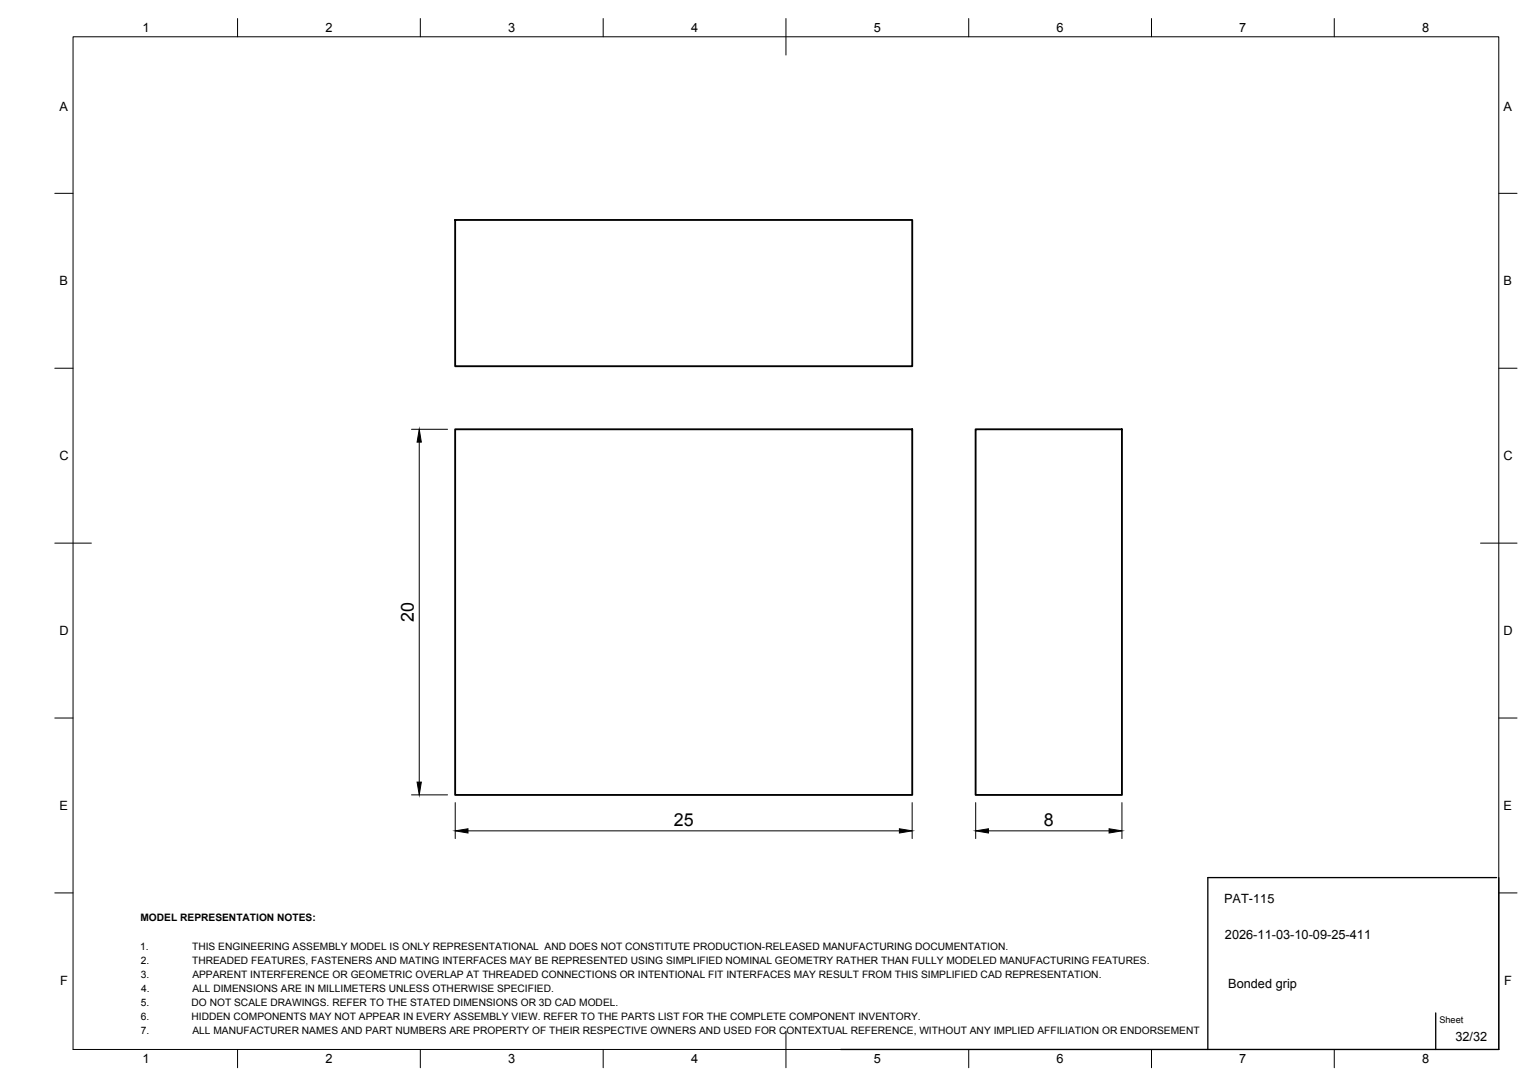
ISO-10303-21;
HEADER;
/* Generated by software containing ST-Developer
 * from STEP Tools, Inc. (www.steptools.com) 
 */

FILE_DESCRIPTION(
/* description */ ('Union bypass pipe loop'),
/* implementation_level */ '2;1');

FILE_NAME(
/* name */ 'Bonded grip.step',
/* time_stamp */ '2026-10-27T21:00:29-07:00',
/* author */ (''),
/* organization */ (''),
/* preprocessor_version */ 'ST-DEVELOPER v20.2',
/* originating_system */ 'Autodesk Translation Framework v15.17.0.0',
/* authorisation */ '');

FILE_SCHEMA (('AUTOMOTIVE_DESIGN { 1 0 10303 214 3 1 1 }'));
ENDSEC;

DATA;
#10=MECHANICAL_DESIGN_GEOMETRIC_PRESENTATION_REPRESENTATION('',(#475),#10095);
#411=SHAPE_REPRESENTATION_RELATIONSHIP('SRR','None',#10281,#443);
#443=ADVANCED_BREP_SHAPE_REPRESENTATION('',(#504),#10093);
#475=STYLED_ITEM('',(#10507),#504);
#504=MANIFOLD_SOLID_BREP('Body1',#5549);
#818=PLANE('',#6581);
#819=PLANE('',#6582);
#820=PLANE('',#6583);
#821=PLANE('',#6584);
#822=PLANE('',#6585);
#823=PLANE('',#6586);
#1145=FACE_OUTER_BOUND('',#1600,.T.);
#1146=FACE_OUTER_BOUND('',#1601,.T.);
#1147=FACE_OUTER_BOUND('',#1602,.T.);
#1148=FACE_OUTER_BOUND('',#1603,.T.);
#1149=FACE_OUTER_BOUND('',#1604,.T.);
#1150=FACE_OUTER_BOUND('',#1605,.T.);
#1600=EDGE_LOOP('',(#4996,#4997,#4998,#4999));
#1601=EDGE_LOOP('',(#5000,#5001,#5002,#5003));
#1602=EDGE_LOOP('',(#5004,#5005,#5006,#5007));
#1603=EDGE_LOOP('',(#5008,#5009,#5010,#5011));
#1604=EDGE_LOOP('',(#5012,#5013,#5014,#5015));
#1605=EDGE_LOOP('',(#5016,#5017,#5018,#5019));
#1964=LINE('',#9925,#2340);
#1965=LINE('',#9927,#2341);
#1966=LINE('',#9929,#2342);
#1967=LINE('',#9930,#2343);
#1968=LINE('',#9933,#2344);
#1969=LINE('',#9935,#2345);
#1970=LINE('',#9936,#2346);
#1971=LINE('',#9939,#2347);
#1972=LINE('',#9941,#2348);
#1973=LINE('',#9942,#2349);
#1974=LINE('',#9944,#2350);
#1975=LINE('',#9945,#2351);
#2340=VECTOR('',#8314,1.);
#2341=VECTOR('',#8315,1.);
#2342=VECTOR('',#8316,1.);
#2343=VECTOR('',#8317,1.);
#2344=VECTOR('',#8320,1.);
#2345=VECTOR('',#8321,1.);
#2346=VECTOR('',#8322,1.);
#2347=VECTOR('',#8325,1.);
#2348=VECTOR('',#8326,1.);
#2349=VECTOR('',#8327,1.);
#2350=VECTOR('',#8330,1.);
#2351=VECTOR('',#8331,1.);
#3040=VERTEX_POINT('',#9923);
#3041=VERTEX_POINT('',#9924);
#3042=VERTEX_POINT('',#9926);
#3043=VERTEX_POINT('',#9928);
#3044=VERTEX_POINT('',#9932);
#3045=VERTEX_POINT('',#9934);
#3046=VERTEX_POINT('',#9938);
#3047=VERTEX_POINT('',#9940);
#3696=EDGE_CURVE('',#3040,#3041,#1964,.T.);
#3697=EDGE_CURVE('',#3041,#3042,#1965,.T.);
#3698=EDGE_CURVE('',#3043,#3042,#1966,.T.);
#3699=EDGE_CURVE('',#3040,#3043,#1967,.T.);
#3700=EDGE_CURVE('',#3044,#3040,#1968,.T.);
#3701=EDGE_CURVE('',#3045,#3043,#1969,.T.);
#3702=EDGE_CURVE('',#3044,#3045,#1970,.T.);
#3703=EDGE_CURVE('',#3046,#3044,#1971,.T.);
#3704=EDGE_CURVE('',#3047,#3045,#1972,.T.);
#3705=EDGE_CURVE('',#3046,#3047,#1973,.T.);
#3706=EDGE_CURVE('',#3041,#3046,#1974,.T.);
#3707=EDGE_CURVE('',#3042,#3047,#1975,.T.);
#4996=ORIENTED_EDGE('',*,*,#3696,.T.);
#4997=ORIENTED_EDGE('',*,*,#3697,.T.);
#4998=ORIENTED_EDGE('',*,*,#3698,.F.);
#4999=ORIENTED_EDGE('',*,*,#3699,.F.);
#5000=ORIENTED_EDGE('',*,*,#3700,.T.);
#5001=ORIENTED_EDGE('',*,*,#3699,.T.);
#5002=ORIENTED_EDGE('',*,*,#3701,.F.);
#5003=ORIENTED_EDGE('',*,*,#3702,.F.);
#5004=ORIENTED_EDGE('',*,*,#3703,.T.);
#5005=ORIENTED_EDGE('',*,*,#3702,.T.);
#5006=ORIENTED_EDGE('',*,*,#3704,.F.);
#5007=ORIENTED_EDGE('',*,*,#3705,.F.);
#5008=ORIENTED_EDGE('',*,*,#3706,.T.);
#5009=ORIENTED_EDGE('',*,*,#3705,.T.);
#5010=ORIENTED_EDGE('',*,*,#3707,.F.);
#5011=ORIENTED_EDGE('',*,*,#3697,.F.);
#5012=ORIENTED_EDGE('',*,*,#3707,.T.);
#5013=ORIENTED_EDGE('',*,*,#3704,.T.);
#5014=ORIENTED_EDGE('',*,*,#3701,.T.);
#5015=ORIENTED_EDGE('',*,*,#3698,.T.);
#5016=ORIENTED_EDGE('',*,*,#3706,.F.);
#5017=ORIENTED_EDGE('',*,*,#3696,.F.);
#5018=ORIENTED_EDGE('',*,*,#3700,.F.);
#5019=ORIENTED_EDGE('',*,*,#3703,.F.);
#5494=ADVANCED_FACE('',(#1145),#818,.T.);
#5495=ADVANCED_FACE('',(#1146),#819,.T.);
#5496=ADVANCED_FACE('',(#1147),#820,.T.);
#5497=ADVANCED_FACE('',(#1148),#821,.T.);
#5498=ADVANCED_FACE('',(#1149),#822,.T.);
#5499=ADVANCED_FACE('',(#1150),#823,.F.);
#5549=CLOSED_SHELL('',(#5494,#5495,#5496,#5497,#5498,#5499));
#6580=AXIS2_PLACEMENT_3D('',#9921,#8310,#8311);
#6581=AXIS2_PLACEMENT_3D('',#9922,#8312,#8313);
#6582=AXIS2_PLACEMENT_3D('',#9931,#8318,#8319);
#6583=AXIS2_PLACEMENT_3D('',#9937,#8323,#8324);
#6584=AXIS2_PLACEMENT_3D('',#9943,#8328,#8329);
#6585=AXIS2_PLACEMENT_3D('',#9946,#8332,#8333);
#6586=AXIS2_PLACEMENT_3D('',#9947,#8334,#8335);
#8310=DIRECTION('axis',(0.,0.,1.));
#8311=DIRECTION('refdir',(1.,0.,0.));
#8312=DIRECTION('center_axis',(0.,1.,0.));
#8313=DIRECTION('ref_axis',(-1.,0.,0.));
#8314=DIRECTION('',(-1.,0.,0.));
#8315=DIRECTION('',(0.,0.,1.));
#8316=DIRECTION('',(-1.,0.,0.));
#8317=DIRECTION('',(0.,0.,1.));
#8318=DIRECTION('center_axis',(1.,0.,0.));
#8319=DIRECTION('ref_axis',(0.,1.,0.));
#8320=DIRECTION('',(0.,1.,0.));
#8321=DIRECTION('',(0.,1.,0.));
#8322=DIRECTION('',(0.,0.,1.));
#8323=DIRECTION('center_axis',(0.,-1.,0.));
#8324=DIRECTION('ref_axis',(1.,0.,0.));
#8325=DIRECTION('',(1.,0.,0.));
#8326=DIRECTION('',(1.,0.,0.));
#8327=DIRECTION('',(0.,0.,1.));
#8328=DIRECTION('center_axis',(-1.,0.,0.));
#8329=DIRECTION('ref_axis',(0.,-1.,0.));
#8330=DIRECTION('',(0.,-1.,0.));
#8331=DIRECTION('',(0.,-1.,0.));
#8332=DIRECTION('center_axis',(0.,0.,1.));
#8333=DIRECTION('ref_axis',(1.,0.,0.));
#8334=DIRECTION('center_axis',(0.,0.,1.));
#8335=DIRECTION('ref_axis',(1.,0.,0.));
#9921=CARTESIAN_POINT('',(0.,0.,0.));
#9922=CARTESIAN_POINT('Origin',(8.5,1.,9.4));
#9923=CARTESIAN_POINT('',(8.5,1.,9.4));
#9924=CARTESIAN_POINT('',(6.,1.,9.4));
#9925=CARTESIAN_POINT('',(8.5,1.,9.4));
#9926=CARTESIAN_POINT('',(6.,1.,10.2));
#9927=CARTESIAN_POINT('',(6.,1.,9.4));
#9928=CARTESIAN_POINT('',(8.5,1.,10.2));
#9929=CARTESIAN_POINT('',(8.5,1.,10.2));
#9930=CARTESIAN_POINT('',(8.5,1.,9.4));
#9931=CARTESIAN_POINT('Origin',(8.5,-1.,9.4));
#9932=CARTESIAN_POINT('',(8.5,-1.,9.4));
#9933=CARTESIAN_POINT('',(8.5,-1.,9.4));
#9934=CARTESIAN_POINT('',(8.5,-1.,10.2));
#9935=CARTESIAN_POINT('',(8.5,-1.,10.2));
#9936=CARTESIAN_POINT('',(8.5,-1.,9.4));
#9937=CARTESIAN_POINT('Origin',(6.,-1.,9.4));
#9938=CARTESIAN_POINT('',(6.,-1.,9.4));
#9939=CARTESIAN_POINT('',(6.,-1.,9.4));
#9940=CARTESIAN_POINT('',(6.,-1.,10.2));
#9941=CARTESIAN_POINT('',(6.,-1.,10.2));
#9942=CARTESIAN_POINT('',(6.,-1.,9.4));
#9943=CARTESIAN_POINT('Origin',(6.,1.,9.4));
#9944=CARTESIAN_POINT('',(6.,1.,9.4));
#9945=CARTESIAN_POINT('',(6.,1.,10.2));
#9946=CARTESIAN_POINT('Origin',(7.25,0.,10.2));
#9947=CARTESIAN_POINT('Origin',(7.25,0.,9.4));
#10056=UNCERTAINTY_MEASURE_WITH_UNIT(LENGTH_MEASURE(0.001),#10096,
'DISTANCE_ACCURACY_VALUE',
'Maximum model space distance between geometric entities at asserted c
onnectivities');
#10058=UNCERTAINTY_MEASURE_WITH_UNIT(LENGTH_MEASURE(0.001),#10096,
'DISTANCE_ACCURACY_VALUE',
'Maximum model space distance between geometric entities at asserted c
onnectivities');
#10093=(
GEOMETRIC_REPRESENTATION_CONTEXT(3)
GLOBAL_UNCERTAINTY_ASSIGNED_CONTEXT((#10056))
GLOBAL_UNIT_ASSIGNED_CONTEXT((#10096,#10098,#10099))
REPRESENTATION_CONTEXT('','3D')
);
#10095=(
GEOMETRIC_REPRESENTATION_CONTEXT(3)
GLOBAL_UNCERTAINTY_ASSIGNED_CONTEXT((#10058))
GLOBAL_UNIT_ASSIGNED_CONTEXT((#10096,#10098,#10099))
REPRESENTATION_CONTEXT('','3D')
);
#10096=(
LENGTH_UNIT()
NAMED_UNIT(*)
SI_UNIT(.CENTI.,.METRE.)
);
#10098=(
NAMED_UNIT(*)
PLANE_ANGLE_UNIT()
SI_UNIT($,.RADIAN.)
);
#10099=(
NAMED_UNIT(*)
SI_UNIT($,.STERADIAN.)
SOLID_ANGLE_UNIT()
);
#10134=SHAPE_DEFINITION_REPRESENTATION(#10237,#10281);
#10237=PRODUCT_DEFINITION_SHAPE('',$,#10318);
#10281=SHAPE_REPRESENTATION('',(#6580),#10093);
#10283=PRODUCT_DEFINITION_CONTEXT('part definition',#10393,'design');
#10318=PRODUCT_DEFINITION('Bonded grip','Bonded grip',#10354,#10283);
#10354=PRODUCT_DEFINITION_FORMATION('',$,#10429);
#10393=APPLICATION_CONTEXT(
'Core Data for Automotive Mechanical Design Process');
#10394=PRODUCT_CONTEXT('part definition',#10393,'mechanical');
#10429=PRODUCT('Bonded grip','Bonded grip','Bonded grip',(#10394));
#10501=COLOUR_RGB('Black',0.12,0.14,0.17);
#10502=FILL_AREA_STYLE_COLOUR('',#10501);
#10503=FILL_AREA_STYLE('',(#10502));
#10504=SURFACE_STYLE_FILL_AREA(#10503);
#10505=SURFACE_SIDE_STYLE('',(#10504));
#10506=SURFACE_STYLE_USAGE(.BOTH.,#10505);
#10507=PRESENTATION_STYLE_ASSIGNMENT((#10506));
ENDSEC;
END-ISO-10303-21;
